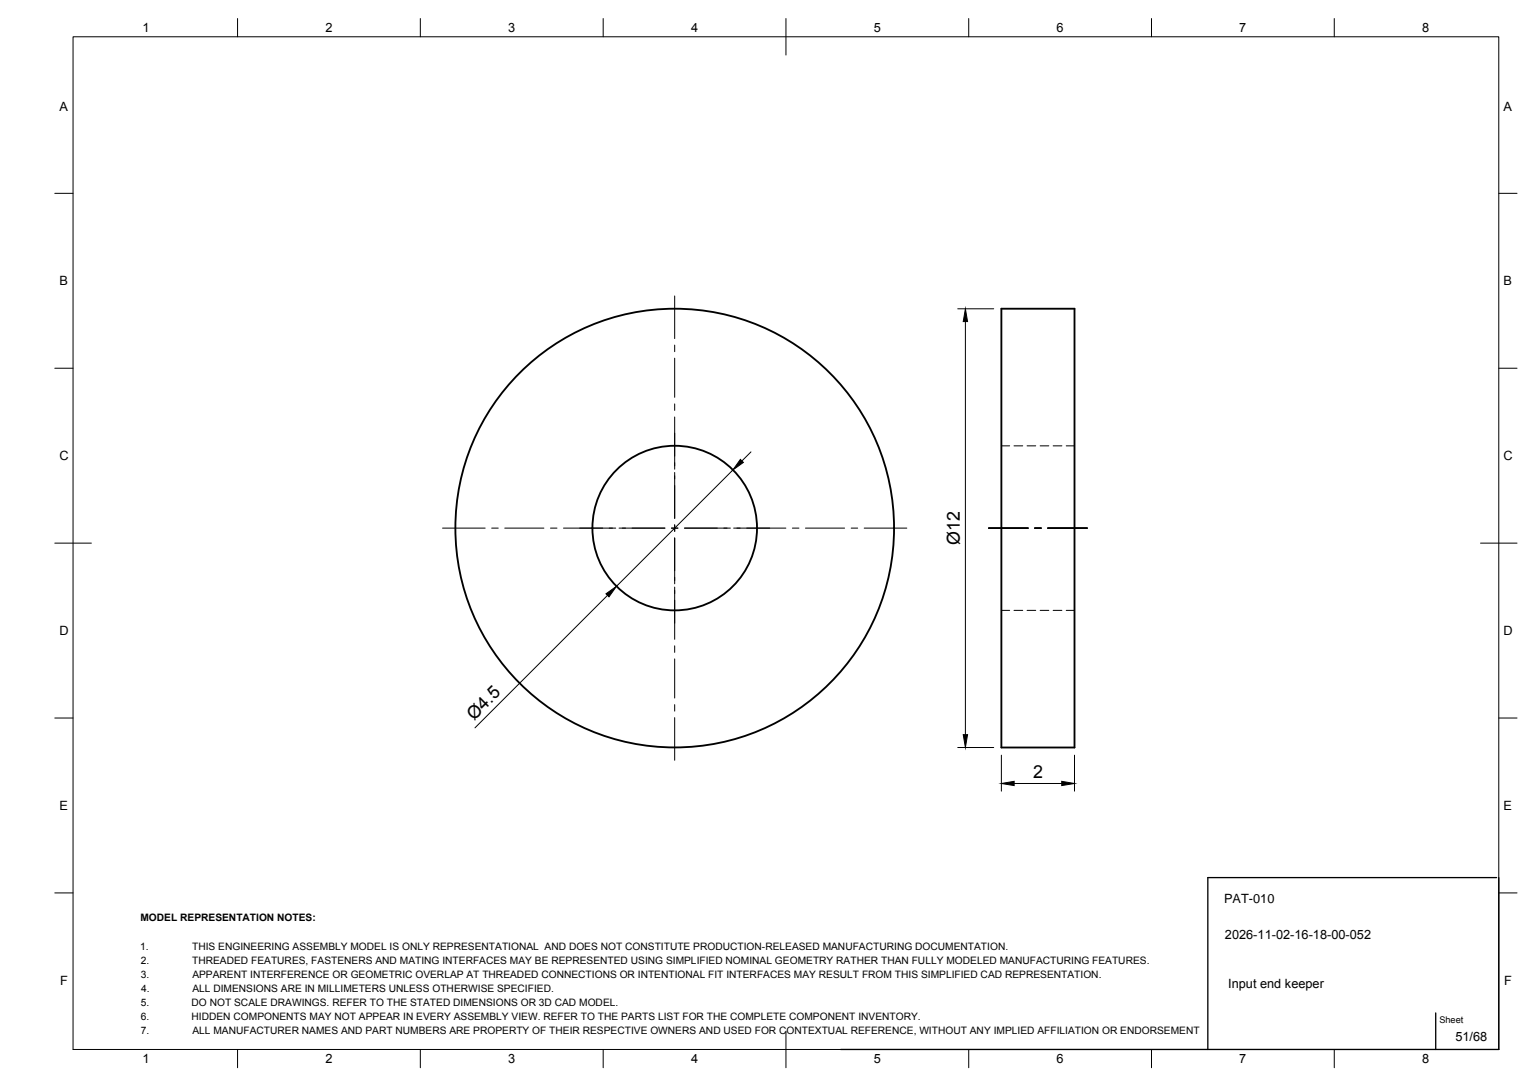
ISO-10303-21;
HEADER;
/* Generated by software containing ST-Developer
 * from STEP Tools, Inc. (www.steptools.com) 
 */

FILE_DESCRIPTION(
/* description */ ('Belt conveyor head drive unit'),
/* implementation_level */ '2;1');

FILE_NAME(
/* name */ 'Input end keeper.step',
/* time_stamp */ '2026-10-28T03:26:19-07:00',
/* author */ (''),
/* organization */ (''),
/* preprocessor_version */ 'ST-DEVELOPER v20.2',
/* originating_system */ 'Autodesk Translation Framework v15.17.0.0',
/* authorisation */ '');

FILE_SCHEMA (('AUTOMOTIVE_DESIGN { 1 0 10303 214 3 1 1 }'));
ENDSEC;

DATA;
#10=MECHANICAL_DESIGN_GEOMETRIC_PRESENTATION_REPRESENTATION('',(#912),#27069);
#758=SHAPE_REPRESENTATION_RELATIONSHIP('SRR','None',#27406,#827);
#827=ADVANCED_BREP_SHAPE_REPRESENTATION('',(#993),#27048);
#912=STYLED_ITEM('',(#27790),#993);
#993=MANIFOLD_SOLID_BREP('Body1',#13781);
#1214=FACE_BOUND('',#3179,.T.);
#1215=FACE_BOUND('',#3181,.T.);
#1556=PLANE('',#15700);
#1557=PLANE('',#15701);
#2174=FACE_OUTER_BOUND('',#3176,.T.);
#2175=FACE_OUTER_BOUND('',#3177,.T.);
#2176=FACE_OUTER_BOUND('',#3178,.T.);
#2177=FACE_OUTER_BOUND('',#3180,.T.);
#3176=EDGE_LOOP('',(#11232,#11233,#11234,#11235));
#3177=EDGE_LOOP('',(#11236,#11237,#11238,#11239));
#3178=EDGE_LOOP('',(#11240));
#3179=EDGE_LOOP('',(#11241));
#3180=EDGE_LOOP('',(#11242));
#3181=EDGE_LOOP('',(#11243));
#4056=LINE('',#24538,#4848);
#4057=LINE('',#24544,#4849);
#4848=VECTOR('',#19260,0.225);
#4849=VECTOR('',#19267,0.6);
#5605=CIRCLE('',#15695,0.225);
#5606=CIRCLE('',#15696,0.225);
#5607=CIRCLE('',#15698,0.6);
#5608=CIRCLE('',#15699,0.6);
#6731=VERTEX_POINT('',#24535);
#6732=VERTEX_POINT('',#24537);
#6733=VERTEX_POINT('',#24541);
#6734=VERTEX_POINT('',#24543);
#8308=EDGE_CURVE('',#6731,#6731,#5605,.T.);
#8309=EDGE_CURVE('',#6731,#6732,#4056,.T.);
#8310=EDGE_CURVE('',#6732,#6732,#5606,.T.);
#8311=EDGE_CURVE('',#6733,#6733,#5607,.T.);
#8312=EDGE_CURVE('',#6733,#6734,#4057,.T.);
#8313=EDGE_CURVE('',#6734,#6734,#5608,.T.);
#11232=ORIENTED_EDGE('',*,*,#8308,.F.);
#11233=ORIENTED_EDGE('',*,*,#8309,.T.);
#11234=ORIENTED_EDGE('',*,*,#8310,.T.);
#11235=ORIENTED_EDGE('',*,*,#8309,.F.);
#11236=ORIENTED_EDGE('',*,*,#8311,.F.);
#11237=ORIENTED_EDGE('',*,*,#8312,.T.);
#11238=ORIENTED_EDGE('',*,*,#8313,.T.);
#11239=ORIENTED_EDGE('',*,*,#8312,.F.);
#11240=ORIENTED_EDGE('',*,*,#8311,.T.);
#11241=ORIENTED_EDGE('',*,*,#8308,.T.);
#11242=ORIENTED_EDGE('',*,*,#8313,.F.);
#11243=ORIENTED_EDGE('',*,*,#8310,.F.);
#12736=CYLINDRICAL_SURFACE('',#15694,0.225);
#12737=CYLINDRICAL_SURFACE('',#15697,0.6);
#13453=ADVANCED_FACE('',(#2174),#12736,.F.);
#13454=ADVANCED_FACE('',(#2175),#12737,.T.);
#13455=ADVANCED_FACE('',(#2176,#1214),#1556,.T.);
#13456=ADVANCED_FACE('',(#2177,#1215),#1557,.F.);
#13781=CLOSED_SHELL('',(#13453,#13454,#13455,#13456));
#15693=AXIS2_PLACEMENT_3D('',#24533,#19254,#19255);
#15694=AXIS2_PLACEMENT_3D('',#24534,#19256,#19257);
#15695=AXIS2_PLACEMENT_3D('',#24536,#19258,#19259);
#15696=AXIS2_PLACEMENT_3D('',#24539,#19261,#19262);
#15697=AXIS2_PLACEMENT_3D('',#24540,#19263,#19264);
#15698=AXIS2_PLACEMENT_3D('',#24542,#19265,#19266);
#15699=AXIS2_PLACEMENT_3D('',#24545,#19268,#19269);
#15700=AXIS2_PLACEMENT_3D('',#24546,#19270,#19271);
#15701=AXIS2_PLACEMENT_3D('',#24547,#19272,#19273);
#19254=DIRECTION('axis',(0.,0.,1.));
#19255=DIRECTION('refdir',(1.,0.,0.));
#19256=DIRECTION('center_axis',(0.,1.,0.));
#19257=DIRECTION('ref_axis',(1.,0.,0.));
#19258=DIRECTION('center_axis',(0.,-1.,0.));
#19259=DIRECTION('ref_axis',(1.,0.,0.));
#19260=DIRECTION('',(0.,-1.,0.));
#19261=DIRECTION('center_axis',(0.,-1.,0.));
#19262=DIRECTION('ref_axis',(1.,0.,0.));
#19263=DIRECTION('center_axis',(0.,1.,0.));
#19264=DIRECTION('ref_axis',(1.,0.,0.));
#19265=DIRECTION('center_axis',(0.,1.,0.));
#19266=DIRECTION('ref_axis',(1.,0.,0.));
#19267=DIRECTION('',(0.,-1.,0.));
#19268=DIRECTION('center_axis',(0.,1.,0.));
#19269=DIRECTION('ref_axis',(1.,0.,0.));
#19270=DIRECTION('center_axis',(0.,1.,0.));
#19271=DIRECTION('ref_axis',(1.,0.,0.));
#19272=DIRECTION('center_axis',(0.,1.,0.));
#19273=DIRECTION('ref_axis',(1.,0.,0.));
#24533=CARTESIAN_POINT('',(0.,0.,0.));
#24534=CARTESIAN_POINT('Origin',(0.,-5.2,7.));
#24535=CARTESIAN_POINT('',(-0.225,-5.,7.));
#24536=CARTESIAN_POINT('Origin',(0.,-5.,7.));
#24537=CARTESIAN_POINT('',(-0.225,-5.2,7.));
#24538=CARTESIAN_POINT('',(-0.225,-5.2,7.));
#24539=CARTESIAN_POINT('Origin',(0.,-5.2,7.));
#24540=CARTESIAN_POINT('Origin',(0.,-5.2,7.));
#24541=CARTESIAN_POINT('',(-0.6,-5.,7.));
#24542=CARTESIAN_POINT('Origin',(0.,-5.,7.));
#24543=CARTESIAN_POINT('',(-0.6,-5.2,7.));
#24544=CARTESIAN_POINT('',(-0.6,-5.2,7.));
#24545=CARTESIAN_POINT('Origin',(0.,-5.2,7.));
#24546=CARTESIAN_POINT('Origin',(0.,-5.,7.));
#24547=CARTESIAN_POINT('Origin',(0.,-5.2,7.));
#26971=UNCERTAINTY_MEASURE_WITH_UNIT(LENGTH_MEASURE(0.001),#27070,
'DISTANCE_ACCURACY_VALUE',
'Maximum model space distance between geometric entities at asserted c
onnectivities');
#26992=UNCERTAINTY_MEASURE_WITH_UNIT(LENGTH_MEASURE(0.001),#27070,
'DISTANCE_ACCURACY_VALUE',
'Maximum model space distance between geometric entities at asserted c
onnectivities');
#27048=(
GEOMETRIC_REPRESENTATION_CONTEXT(3)
GLOBAL_UNCERTAINTY_ASSIGNED_CONTEXT((#26971))
GLOBAL_UNIT_ASSIGNED_CONTEXT((#27070,#27072,#27073))
REPRESENTATION_CONTEXT('','3D')
);
#27069=(
GEOMETRIC_REPRESENTATION_CONTEXT(3)
GLOBAL_UNCERTAINTY_ASSIGNED_CONTEXT((#26992))
GLOBAL_UNIT_ASSIGNED_CONTEXT((#27070,#27072,#27073))
REPRESENTATION_CONTEXT('','3D')
);
#27070=(
LENGTH_UNIT()
NAMED_UNIT(*)
SI_UNIT(.CENTI.,.METRE.)
);
#27072=(
NAMED_UNIT(*)
PLANE_ANGLE_UNIT()
SI_UNIT($,.RADIAN.)
);
#27073=(
NAMED_UNIT(*)
SI_UNIT($,.STERADIAN.)
SOLID_ANGLE_UNIT()
);
#27129=SHAPE_DEFINITION_REPRESENTATION(#27217,#27406);
#27217=PRODUCT_DEFINITION_SHAPE('',$,#27483);
#27406=SHAPE_REPRESENTATION('',(#15693),#27048);
#27427=PRODUCT_DEFINITION_CONTEXT('part definition',#27657,'design');
#27483=PRODUCT_DEFINITION('Input end keeper','Input end keeper',#27559,
#27427);
#27559=PRODUCT_DEFINITION_FORMATION('',$,#27714);
#27657=APPLICATION_CONTEXT(
'Core Data for Automotive Mechanical Design Process');
#27658=PRODUCT_CONTEXT('part definition',#27657,'mechanical');
#27714=PRODUCT('Input end keeper','Input end keeper','Input end keeper',
(#27658));
#27784=COLOUR_RGB('Sky Blue',0.24,0.69,0.87);
#27785=FILL_AREA_STYLE_COLOUR('',#27784);
#27786=FILL_AREA_STYLE('',(#27785));
#27787=SURFACE_STYLE_FILL_AREA(#27786);
#27788=SURFACE_SIDE_STYLE('',(#27787));
#27789=SURFACE_STYLE_USAGE(.BOTH.,#27788);
#27790=PRESENTATION_STYLE_ASSIGNMENT((#27789));
ENDSEC;
END-ISO-10303-21;
